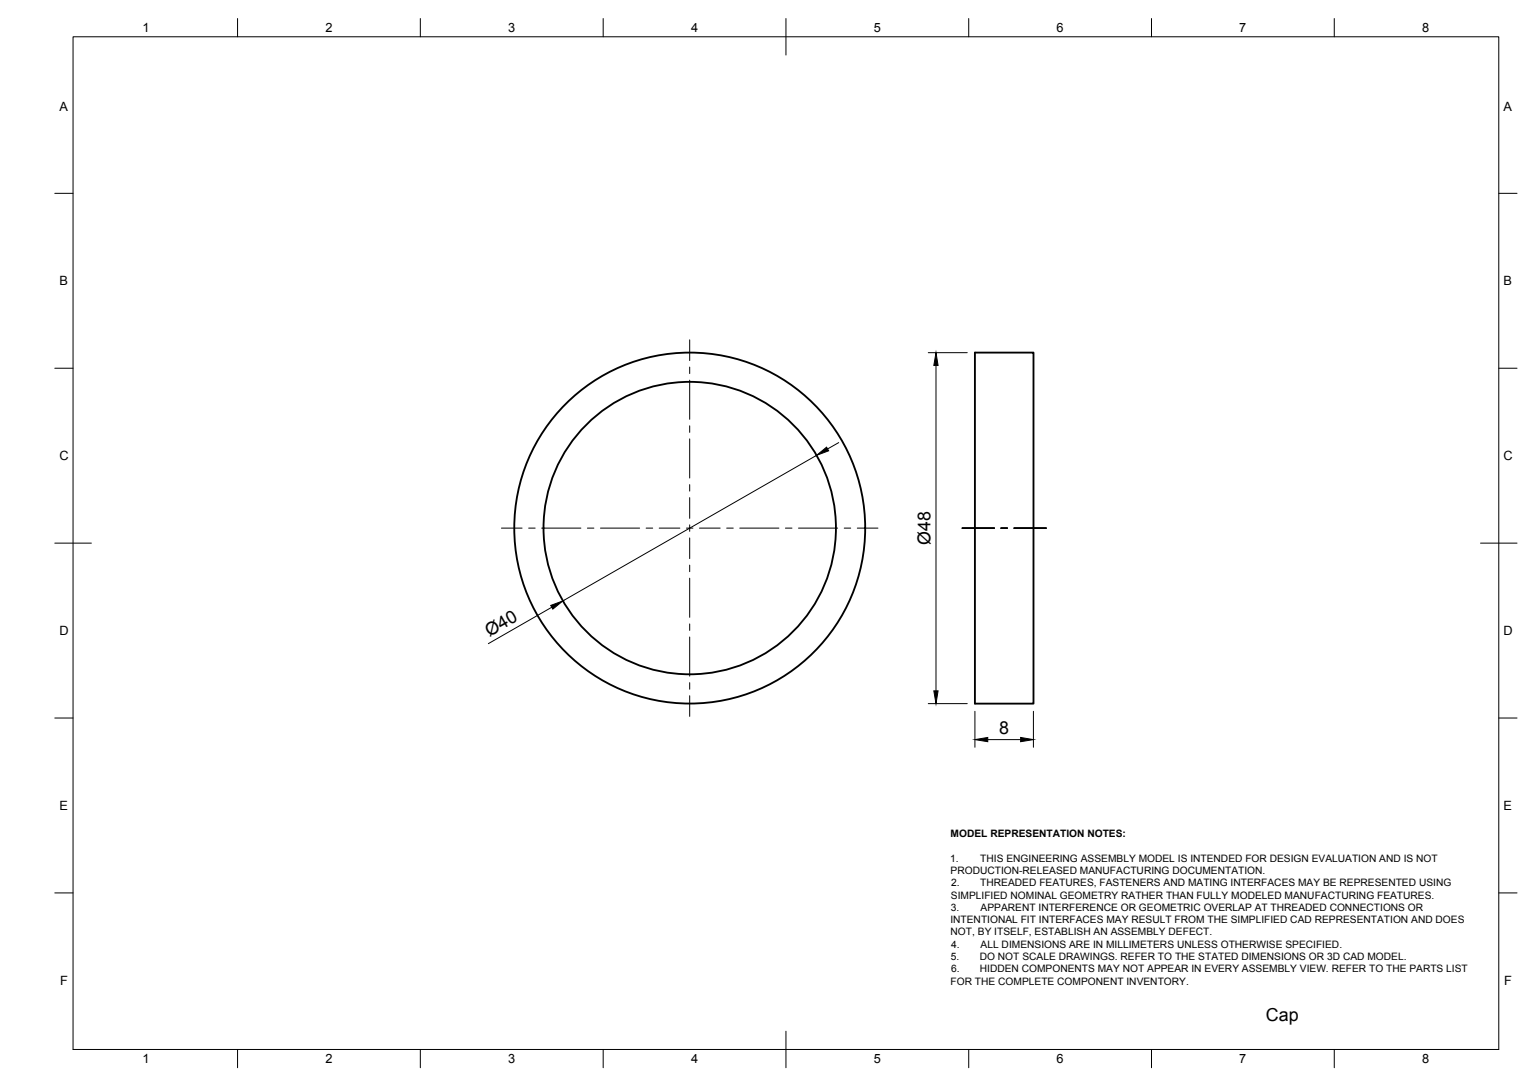
ISO-10303-21;
HEADER;
/* Generated by software containing ST-Developer
 * from STEP Tools, Inc. (www.steptools.com) 
 */

FILE_DESCRIPTION(
/* description */ (''),
/* implementation_level */ '2;1');

FILE_NAME(
/* name */ 'Cap.step',
/* time_stamp */ '2026-10-06T13:31:15-07:00',
/* author */ (''),
/* organization */ (''),
/* preprocessor_version */ 'ST-DEVELOPER v20.2',
/* originating_system */ 'Autodesk Translation Framework v15.15.0.0',
/* authorisation */ '');

FILE_SCHEMA (('AUTOMOTIVE_DESIGN { 1 0 10303 214 3 1 1 }'));
ENDSEC;

DATA;
#10=MECHANICAL_DESIGN_GEOMETRIC_PRESENTATION_REPRESENTATION('',(#80),#3154);
#62=SHAPE_REPRESENTATION_RELATIONSHIP('SRR','None',#3190,#71);
#71=ADVANCED_BREP_SHAPE_REPRESENTATION('',(#89),#3146);
#80=STYLED_ITEM('',(#3243),#89);
#89=MANIFOLD_SOLID_BREP('Body1',#1082);
#99=PLANE('',#1203);
#100=PLANE('',#1210);
#101=PLANE('',#1211);
#132=FACE_BOUND('',#245,.T.);
#143=CIRCLE('',#1204,20.);
#144=CIRCLE('',#1206,20.);
#145=CIRCLE('',#1208,24.);
#146=CIRCLE('',#1209,24.);
#177=FACE_OUTER_BOUND('',#240,.T.);
#178=FACE_OUTER_BOUND('',#241,.T.);
#179=FACE_OUTER_BOUND('',#242,.T.);
#180=FACE_OUTER_BOUND('',#243,.T.);
#181=FACE_OUTER_BOUND('',#244,.T.);
#240=EDGE_LOOP('',(#760));
#241=EDGE_LOOP('',(#761,#762,#763,#764));
#242=EDGE_LOOP('',(#765,#766,#767,#768));
#243=EDGE_LOOP('',(#769));
#244=EDGE_LOOP('',(#770));
#245=EDGE_LOOP('',(#771));
#306=LINE('',#1732,#372);
#307=LINE('',#1738,#373);
#372=VECTOR('',#1324,20.);
#373=VECTOR('',#1331,24.);
#492=VERTEX_POINT('',#1728);
#493=VERTEX_POINT('',#1731);
#494=VERTEX_POINT('',#1735);
#495=VERTEX_POINT('',#1737);
#596=EDGE_CURVE('',#492,#492,#143,.T.);
#597=EDGE_CURVE('',#492,#493,#306,.T.);
#598=EDGE_CURVE('',#493,#493,#144,.T.);
#599=EDGE_CURVE('',#494,#494,#145,.T.);
#600=EDGE_CURVE('',#494,#495,#307,.T.);
#601=EDGE_CURVE('',#495,#495,#146,.T.);
#760=ORIENTED_EDGE('',*,*,#596,.F.);
#761=ORIENTED_EDGE('',*,*,#596,.T.);
#762=ORIENTED_EDGE('',*,*,#597,.T.);
#763=ORIENTED_EDGE('',*,*,#598,.F.);
#764=ORIENTED_EDGE('',*,*,#597,.F.);
#765=ORIENTED_EDGE('',*,*,#599,.F.);
#766=ORIENTED_EDGE('',*,*,#600,.T.);
#767=ORIENTED_EDGE('',*,*,#601,.F.);
#768=ORIENTED_EDGE('',*,*,#600,.F.);
#769=ORIENTED_EDGE('',*,*,#601,.T.);
#770=ORIENTED_EDGE('',*,*,#599,.T.);
#771=ORIENTED_EDGE('',*,*,#598,.T.);
#1012=CYLINDRICAL_SURFACE('',#1205,20.);
#1013=CYLINDRICAL_SURFACE('',#1207,24.);
#1028=ADVANCED_FACE('',(#177),#99,.F.);
#1029=ADVANCED_FACE('',(#178),#1012,.F.);
#1030=ADVANCED_FACE('',(#179),#1013,.T.);
#1031=ADVANCED_FACE('',(#180),#100,.T.);
#1032=ADVANCED_FACE('',(#181,#132),#101,.F.);
#1082=CLOSED_SHELL('',(#1028,#1029,#1030,#1031,#1032));
#1202=AXIS2_PLACEMENT_3D('',#1726,#1316,#1317);
#1203=AXIS2_PLACEMENT_3D('',#1727,#1318,#1319);
#1204=AXIS2_PLACEMENT_3D('',#1729,#1320,#1321);
#1205=AXIS2_PLACEMENT_3D('',#1730,#1322,#1323);
#1206=AXIS2_PLACEMENT_3D('',#1733,#1325,#1326);
#1207=AXIS2_PLACEMENT_3D('',#1734,#1327,#1328);
#1208=AXIS2_PLACEMENT_3D('',#1736,#1329,#1330);
#1209=AXIS2_PLACEMENT_3D('',#1739,#1332,#1333);
#1210=AXIS2_PLACEMENT_3D('',#1740,#1334,#1335);
#1211=AXIS2_PLACEMENT_3D('',#1741,#1336,#1337);
#1316=DIRECTION('axis',(0.,0.,1.));
#1317=DIRECTION('refdir',(1.,0.,0.));
#1318=DIRECTION('center_axis',(0.,0.,-1.));
#1319=DIRECTION('ref_axis',(1.,0.,0.));
#1320=DIRECTION('center_axis',(0.,0.,-1.));
#1321=DIRECTION('ref_axis',(1.,0.,0.));
#1322=DIRECTION('center_axis',(0.,0.,1.));
#1323=DIRECTION('ref_axis',(1.,0.,0.));
#1324=DIRECTION('',(0.,0.,1.));
#1325=DIRECTION('center_axis',(0.,0.,-1.));
#1326=DIRECTION('ref_axis',(1.,0.,0.));
#1327=DIRECTION('center_axis',(0.,0.,1.));
#1328=DIRECTION('ref_axis',(1.,0.,0.));
#1329=DIRECTION('center_axis',(0.,0.,1.));
#1330=DIRECTION('ref_axis',(1.,0.,0.));
#1331=DIRECTION('',(0.,0.,-1.));
#1332=DIRECTION('center_axis',(0.,0.,-1.));
#1333=DIRECTION('ref_axis',(1.,0.,0.));
#1334=DIRECTION('center_axis',(0.,0.,-1.));
#1335=DIRECTION('ref_axis',(1.,0.,0.));
#1336=DIRECTION('center_axis',(0.,0.,-1.));
#1337=DIRECTION('ref_axis',(1.,0.,0.));
#1726=CARTESIAN_POINT('',(0.,0.,0.));
#1727=CARTESIAN_POINT('Origin',(0.,0.,1.));
#1728=CARTESIAN_POINT('',(-20.,2.44929359829471E-15,1.));
#1729=CARTESIAN_POINT('Origin',(0.,0.,1.));
#1730=CARTESIAN_POINT('Origin',(0.,0.,0.));
#1731=CARTESIAN_POINT('',(-20.,2.44929359829471E-15,8.));
#1732=CARTESIAN_POINT('',(-20.,-2.44929359829471E-15,0.));
#1733=CARTESIAN_POINT('Origin',(0.,0.,8.));
#1734=CARTESIAN_POINT('Origin',(0.,0.,0.));
#1735=CARTESIAN_POINT('',(-24.,2.93915231795365E-15,8.));
#1736=CARTESIAN_POINT('Origin',(0.,0.,8.));
#1737=CARTESIAN_POINT('',(-24.,2.93915231795365E-15,0.));
#1738=CARTESIAN_POINT('',(-24.,-2.93915231795365E-15,0.));
#1739=CARTESIAN_POINT('Origin',(0.,0.,0.));
#1740=CARTESIAN_POINT('Origin',(0.,0.,0.));
#1741=CARTESIAN_POINT('Origin',(0.,0.,8.));
#3135=UNCERTAINTY_MEASURE_WITH_UNIT(LENGTH_MEASURE(0.01),#3155,
'DISTANCE_ACCURACY_VALUE',
'Maximum model space distance between geometric entities at asserted c
onnectivities');
#3143=UNCERTAINTY_MEASURE_WITH_UNIT(LENGTH_MEASURE(0.01),#3155,
'DISTANCE_ACCURACY_VALUE',
'Maximum model space distance between geometric entities at asserted c
onnectivities');
#3146=(
GEOMETRIC_REPRESENTATION_CONTEXT(3)
GLOBAL_UNCERTAINTY_ASSIGNED_CONTEXT((#3135))
GLOBAL_UNIT_ASSIGNED_CONTEXT((#3155,#3157,#3158))
REPRESENTATION_CONTEXT('','3D')
);
#3154=(
GEOMETRIC_REPRESENTATION_CONTEXT(3)
GLOBAL_UNCERTAINTY_ASSIGNED_CONTEXT((#3143))
GLOBAL_UNIT_ASSIGNED_CONTEXT((#3155,#3157,#3158))
REPRESENTATION_CONTEXT('','3D')
);
#3155=(
LENGTH_UNIT()
NAMED_UNIT(*)
SI_UNIT(.MILLI.,.METRE.)
);
#3157=(
NAMED_UNIT(*)
PLANE_ANGLE_UNIT()
SI_UNIT($,.RADIAN.)
);
#3158=(
NAMED_UNIT(*)
SI_UNIT($,.STERADIAN.)
SOLID_ANGLE_UNIT()
);
#3161=SHAPE_DEFINITION_REPRESENTATION(#3171,#3190);
#3171=PRODUCT_DEFINITION_SHAPE('',$,#3201);
#3190=SHAPE_REPRESENTATION('',(#1202),#3146);
#3198=PRODUCT_DEFINITION_CONTEXT('part definition',#3230,'design');
#3201=PRODUCT_DEFINITION('Cap','Cap',#3211,#3198);
#3211=PRODUCT_DEFINITION_FORMATION('',$,#3234);
#3230=APPLICATION_CONTEXT(
'Core Data for Automotive Mechanical Design Process');
#3231=PRODUCT_CONTEXT('part definition',#3230,'mechanical');
#3234=PRODUCT('Cap','Cap',$,(#3231));
#3243=PRESENTATION_STYLE_ASSIGNMENT((#3245));
#3245=SURFACE_STYLE_USAGE(.BOTH.,#3247);
#3247=SURFACE_SIDE_STYLE('',(#3249));
#3249=SURFACE_STYLE_FILL_AREA(#3251);
#3251=FILL_AREA_STYLE('Opaque(160,160,160)',(#3253));
#3253=FILL_AREA_STYLE_COLOUR('Opaque(160,160,160)',#3255);
#3255=COLOUR_RGB('Opaque(160,160,160)', 0.09019608, 0.27058824, 0.51372549);
ENDSEC;
END-ISO-10303-21;
